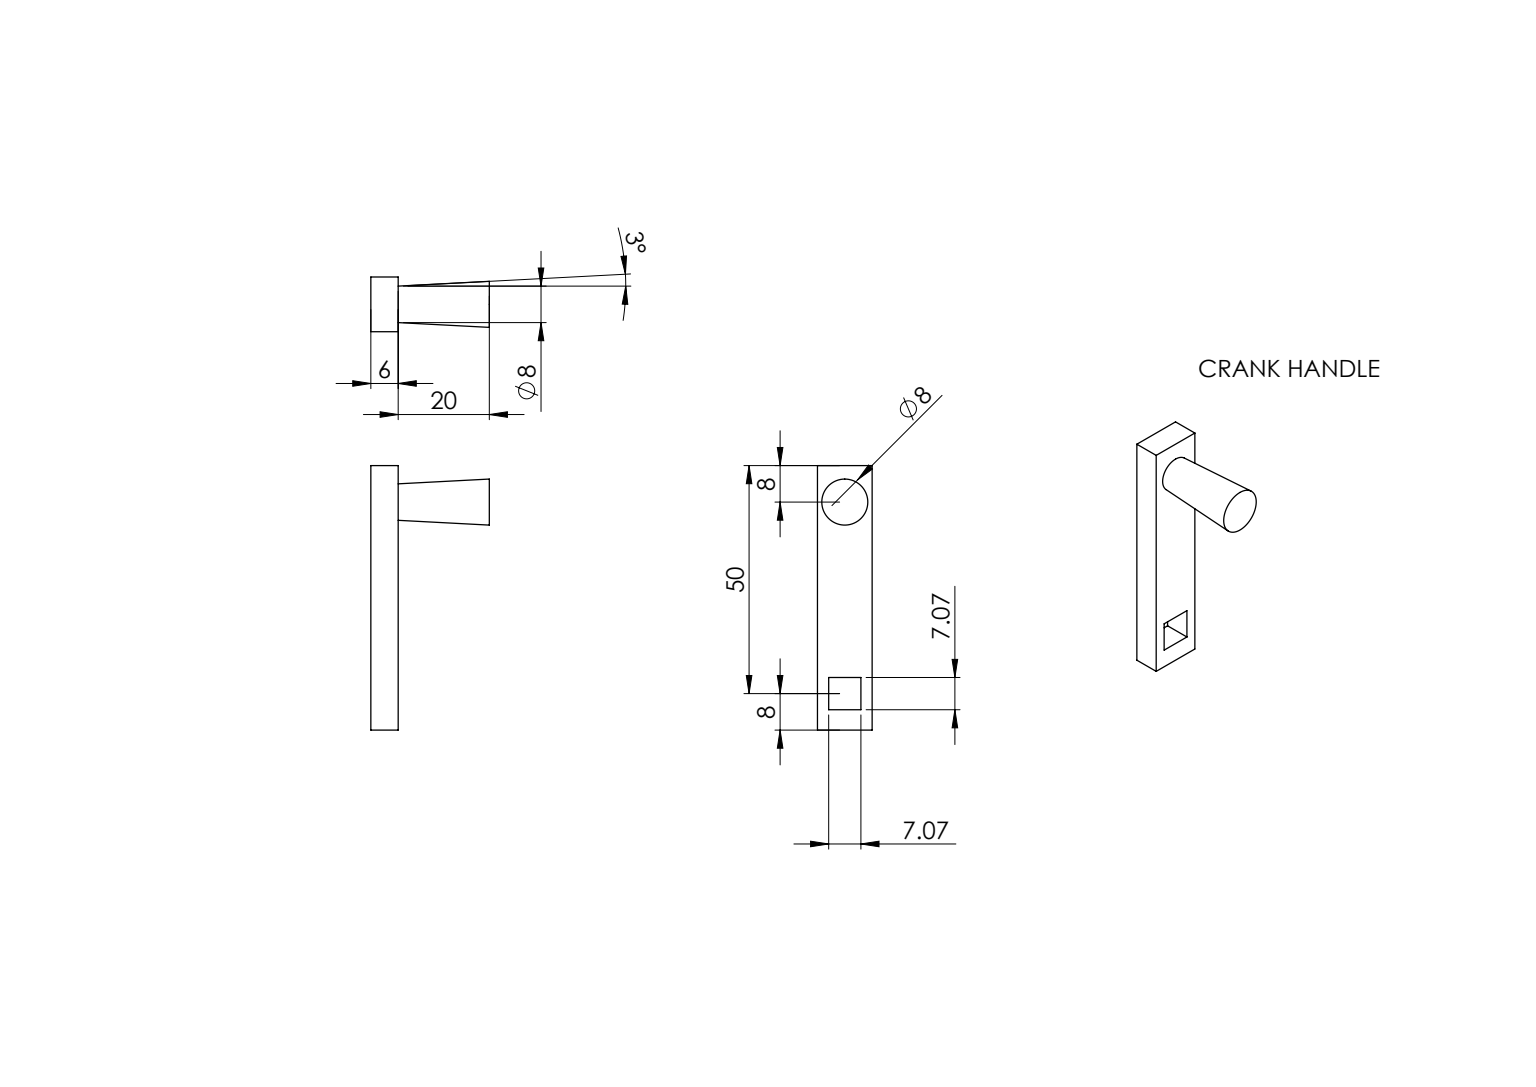
ISO-10303-21;
HEADER;
FILE_DESCRIPTION (('STEP AP214'),
    '1' );
FILE_NAME ('Crank Handle.step',
    '2026-10-22T10:02:39',
    ( '' ),
    ( '' ),
    'SwSTEP 2.0',
    'SolidWorks 2026',
    '' );
FILE_SCHEMA (( 'AUTOMOTIVE_DESIGN' ));
ENDSEC;

DATA;
#15=EDGE_LOOP ( 'NONE', ( #10379, #7375, #3120, #371 ) ) ;
#35=EDGE_CURVE ( 'NONE', #6873, #1790, #10415, .T. ) ;
#58=VECTOR ( 'NONE', #4245, 1000.000000000000000 ) ;
#60=SHAPE_DEFINITION_REPRESENTATION ( #9305, #2176 ) ;
#144=ORIENTED_EDGE ( 'NONE', *, *, #11561, .T. ) ;
#159=AXIS2_PLACEMENT_3D ( 'NONE', #745, #8186, #2789 ) ;
#163=LINE ( 'NONE', #11122, #11282 ) ;
#198=DIRECTION ( 'NONE',  ( 6.033820786006286457E-17, -1.000000000000000000, 0.000000000000000000 ) ) ;
#217=CARTESIAN_POINT ( 'NONE',  ( 47.00000000000000000, 55.00000000000000000, 6.000000000000000000 ) ) ;
#223=DIRECTION ( 'NONE',  ( -1.000000000000000000, -6.033820786006286457E-17, 0.000000000000000000 ) ) ;
#229=CARTESIAN_POINT ( 'NONE',  ( 73.00000000000000000, 91.95184441433917755, -3.614966813601447167E-16 ) ) ;
#242=DIRECTION ( 'NONE',  ( 0.000000000000000000, -0.000000000000000000, 1.000000000000000000 ) ) ;
#271=FACE_OUTER_BOUND ( 'NONE', #5676, .T. ) ;
#301=VERTEX_POINT ( 'NONE', #1190 ) ;
#315=ORIENTED_EDGE ( 'NONE', *, *, #10681, .F. ) ;
#358=ORIENTED_EDGE ( 'NONE', *, *, #7637, .F. ) ;
#371=ORIENTED_EDGE ( 'NONE', *, *, #2057, .T. ) ;
#425=ORIENTED_EDGE ( 'NONE', *, *, #6952, .F. ) ;
#440=DIRECTION ( 'NONE',  ( 0.000000000000000000, 1.000000000000000000, 0.000000000000000000 ) ) ;
#476=LINE ( 'NONE', #4199, #9328 ) ;
#477=STYLED_ITEM ( 'NONE', ( #10437 ), #9416 ) ;
#522=EDGE_CURVE ( 'NONE', #2578, #3782, #9633, .T. ) ;
#579=CARTESIAN_POINT ( 'NONE',  ( 52.99999999999999289, 58.53553390593273065, -3.535533905932738197 ) ) ;
#595=DIRECTION ( 'NONE',  ( 0.000000000000000000, 0.000000000000000000, -1.000000000000000000 ) ) ;
#645=DIRECTION ( 'NONE',  ( 0.000000000000000000, 0.000000000000000000, -1.000000000000000000 ) ) ;
#662=CARTESIAN_POINT ( 'NONE',  ( 53.00000000000000000, 47.00000000000000711, -6.000000000000000000 ) ) ;
#670=UNCERTAINTY_MEASURE_WITH_UNIT (LENGTH_MEASURE( 1.000000000000000082E-05 ), #7474, 'distance_accuracy_value', 'NONE');
#683=ORIENTED_EDGE ( 'NONE', *, *, #522, .T. ) ;
#686=CARTESIAN_POINT ( 'NONE',  ( 47.00000000000000000, 47.00000000000000711, 6.000000000000000000 ) ) ;
#697=DIRECTION ( 'NONE',  ( 0.000000000000000000, 1.000000000000000000, 0.000000000000000000 ) ) ;
#735=DIRECTION ( 'NONE',  ( -0.000000000000000000, -0.000000000000000000, 1.000000000000000000 ) ) ;
#745=CARTESIAN_POINT ( 'NONE',  ( 52.99999999999999289, 97.00000000000000000, -9.797174393178809880E-16 ) ) ;
#779=AXIS2_PLACEMENT_3D ( 'NONE', #3024, #6692, #198 ) ;
#783=( NAMED_UNIT ( * ) PLANE_ANGLE_UNIT ( ) SI_UNIT ( $, .RADIAN. ) );
#840=DIRECTION ( 'NONE',  ( -1.000000000000000000, -6.033820786006286457E-17, -0.000000000000000000 ) ) ;
#922=ORIENTED_EDGE ( 'NONE', *, *, #35, .F. ) ;
#961=VECTOR ( 'NONE', #1461, 1000.000000000000000 ) ;
#980=MANIFOLD_SOLID_BREP ( 'Cavity1', #6172 ) ;
#1018=ORIENTED_EDGE ( 'NONE', *, *, #9096, .F. ) ;
#1060=ORIENTED_EDGE ( 'NONE', *, *, #10956, .T. ) ;
#1092=EDGE_CURVE ( 'NONE', #301, #7726, #4627, .T. ) ;
#1131=ORIENTED_EDGE ( 'NONE', *, *, #4934, .T. ) ;
#1138=ORIENTED_EDGE ( 'NONE', *, *, #8425, .F. ) ;
#1145=LINE ( 'NONE', #7519, #1367 ) ;
#1176=LINE ( 'NONE', #217, #961 ) ;
#1190=CARTESIAN_POINT ( 'NONE',  ( 53.00000000000000000, 105.0000000000000142, -6.000000000000000000 ) ) ;
#1212=FACE_OUTER_BOUND ( 'NONE', #9717, .T. ) ;
#1235=( GEOMETRIC_REPRESENTATION_CONTEXT ( 3 ) GLOBAL_UNCERTAINTY_ASSIGNED_CONTEXT ( ( #3433 ) ) GLOBAL_UNIT_ASSIGNED_CONTEXT ( ( #11335, #6810, #5979 ) ) REPRESENTATION_CONTEXT ( 'NONE', 'WORKASPACE' ) );
#1280=FILL_AREA_STYLE ('',( #9367 ) ) ;
#1281=AXIS2_PLACEMENT_3D ( 'NONE', #8097, #9101, #4381 ) ;
#1335=AXIS2_PLACEMENT_3D ( 'NONE', #3104, #11347, #6769 ) ;
#1367=VECTOR ( 'NONE', #10249, 1000.000000000000000 ) ;
#1383=DIRECTION ( 'NONE',  ( 1.000000000000000000, 0.000000000000000000, 0.000000000000000000 ) ) ;
#1388=ORIENTED_EDGE ( 'NONE', *, *, #7898, .F. ) ;
#1436=DIRECTION ( 'NONE',  ( -1.000000000000000000, -6.033820786006286457E-17, -0.000000000000000000 ) ) ;
#1455=ORIENTED_EDGE ( 'NONE', *, *, #2211, .F. ) ;
#1461=DIRECTION ( 'NONE',  ( 6.033820786006286457E-17, -1.000000000000000000, 0.000000000000000000 ) ) ;
#1473=CARTESIAN_POINT ( 'NONE',  ( 53.00000000000000000, 47.00000000000000711, 0.000000000000000000 ) ) ;
#1476=ORIENTED_EDGE ( 'NONE', *, *, #6323, .T. ) ;
#1582=LINE ( 'NONE', #1637, #9387 ) ;
#1601=CARTESIAN_POINT ( 'NONE',  ( 73.00000000000000000, 97.00000000000000000, -9.797174393178809880E-16 ) ) ;
#1604=PLANE ( 'NONE',  #7645 ) ;
#1637=CARTESIAN_POINT ( 'NONE',  ( 46.99999999999999289, 58.53553390593273065, 3.535533905932731091 ) ) ;
#1734=CARTESIAN_POINT ( 'NONE',  ( 53.00000000000000000, 55.00000000000000000, -6.000000000000000000 ) ) ;
#1746=AXIS2_PLACEMENT_3D ( 'NONE', #8986, #8142, #5448 ) ;
#1756=ADVANCED_FACE ( 'NONE', ( #271 ), #4960, .T. ) ;
#1785=LINE ( 'NONE', #6246, #5721 ) ;
#1790=VERTEX_POINT ( 'NONE', #5026 ) ;
#1835=CONICAL_SURFACE ( 'NONE', #4136, 4.000000000000003553, 0.05235987755983000091 ) ;
#1840=FACE_BOUND ( 'NONE', #1900, .T. ) ;
#1843=DIRECTION ( 'NONE',  ( 6.033820786006286457E-17, -1.000000000000000000, 0.000000000000000000 ) ) ;
#1874=VERTEX_POINT ( 'NONE', #2873 ) ;
#1883=ORIENTED_EDGE ( 'NONE', *, *, #3862, .F. ) ;
#1900=EDGE_LOOP ( 'NONE', ( #3688, #6429 ) ) ;
#1905=PLANE ( 'NONE',  #9512 ) ;
#1938=VECTOR ( 'NONE', #11031, 1000.000000000000000 ) ;
#1956=DIRECTION ( 'NONE',  ( 0.000000000000000000, 1.000000000000000000, 0.000000000000000000 ) ) ;
#1967=CARTESIAN_POINT ( 'NONE',  ( 53.00000000000000000, 105.0000000000000142, 0.000000000000000000 ) ) ;
#1981=ADVANCED_FACE ( 'NONE', ( #9100 ), #7435, .T. ) ;
#2057=EDGE_CURVE ( 'NONE', #7726, #3451, #163, .T. ) ;
#2061=CARTESIAN_POINT ( 'NONE',  ( 53.00000000000000000, 105.0000000000000142, 6.000000000000000000 ) ) ;
#2146=ORIENTED_EDGE ( 'NONE', *, *, #1092, .T. ) ;
#2162=ORIENTED_EDGE ( 'NONE', *, *, #2057, .F. ) ;
#2176=SHAPE_REPRESENTATION ( 'Crank Handle', ( #4738 ), #4498 ) ;
#2211=EDGE_CURVE ( 'NONE', #3782, #1790, #1582, .T. ) ;
#2236=CARTESIAN_POINT ( 'NONE',  ( 53.00000000000000000, 55.00000000000000000, 6.000000000000000000 ) ) ;
#2267=ORIENTED_EDGE ( 'NONE', *, *, #7023, .T. ) ;
#2276=EDGE_CURVE ( 'NONE', #2578, #6873, #3915, .T. ) ;
#2281=MECHANICAL_DESIGN_GEOMETRIC_PRESENTATION_REPRESENTATION('',(#8140),#6886);
#2432=VECTOR ( 'NONE', #8895, 1000.000000000000000 ) ;
#2529=DIRECTION ( 'NONE',  ( -1.000000000000000000, -6.033820786006286457E-17, -0.000000000000000000 ) ) ;
#2576=CARTESIAN_POINT ( 'NONE',  ( 53.00000000000000000, 51.46446609406726935, -3.535533905932738197 ) ) ;
#2578=VERTEX_POINT ( 'NONE', #6201 ) ;
#2622=VECTOR ( 'NONE', #2700, 1000.000000000000114 ) ;
#2666=ORIENTED_EDGE ( 'NONE', *, *, #10956, .F. ) ;
#2680=ORIENTED_EDGE ( 'NONE', *, *, #10681, .T. ) ;
#2697=CARTESIAN_POINT ( 'NONE',  ( 47.00000000000000000, 105.0000000000000142, 0.000000000000000000 ) ) ;
#2700=DIRECTION ( 'NONE',  ( 0.9986295347545739443, 0.05233595624294401505, 0.000000000000000000 ) ) ;
#2748=DIRECTION ( 'NONE',  ( 1.000000000000000000, 6.033820786006286457E-17, 0.000000000000000000 ) ) ;
#2774=EDGE_CURVE ( 'NONE', #9261, #3782, #8383, .T. ) ;
#2789=DIRECTION ( 'NONE',  ( 0.000000000000000000, 1.000000000000000000, 0.000000000000000000 ) ) ;
#2864=AXIS2_PLACEMENT_3D ( 'NONE', #1601, #5268, #697 ) ;
#2870=UNCERTAINTY_MEASURE_WITH_UNIT (LENGTH_MEASURE( 1.000000000000000082E-05 ), #9951, 'distance_accuracy_value', 'NONE');
#2873=CARTESIAN_POINT ( 'NONE',  ( 53.00000000000000000, 51.46446609406726935, 3.535533905932731091 ) ) ;
#2938=ORIENTED_EDGE ( 'NONE', *, *, #6952, .T. ) ;
#3024=CARTESIAN_POINT ( 'NONE',  ( 47.00000000000000000, 2.835895769422954721E-15, 0.000000000000000000 ) ) ;
#3026=SHAPE_REPRESENTATION_RELATIONSHIP ( 'NONE' , 'NONE' ,  #2176, #9416 ) ;
#3080=EDGE_LOOP ( 'NONE', ( #5000, #1476 ) ) ;
#3087=VECTOR ( 'NONE', #2529, 1000.000000000000000 ) ;
#3104=CARTESIAN_POINT ( 'NONE',  ( 53.00000000000000000, 51.46446609406726935, -3.535533905932738197 ) ) ;
#3120=ORIENTED_EDGE ( 'NONE', *, *, #5936, .F. ) ;
#3146=FACE_OUTER_BOUND ( 'NONE', #15, .T. ) ;
#3211=FACE_OUTER_BOUND ( 'NONE', #5333, .T. ) ;
#3280=VERTEX_POINT ( 'NONE', #686 ) ;
#3289=EDGE_LOOP ( 'NONE', ( #1388, #922, #144, #8606 ) ) ;
#3293=VERTEX_POINT ( 'NONE', #8010 ) ;
#3296=CARTESIAN_POINT ( 'NONE',  ( 47.00000000000000000, 51.46446609406726935, -3.535533905932738197 ) ) ;
#3313=CARTESIAN_POINT ( 'NONE',  ( 52.99999999999999289, 93.00000000000000000, -4.256777005095426300E-16 ) ) ;
#3334=CARTESIAN_POINT ( 'NONE',  ( 53.00000000000000000, 47.00000000000000711, 6.000000000000000000 ) ) ;
#3433=UNCERTAINTY_MEASURE_WITH_UNIT (LENGTH_MEASURE( 1.000000000000000082E-05 ), #11335, 'distance_accuracy_value', 'NONE');
#3451=VERTEX_POINT ( 'NONE', #7408 ) ;
#3536=ORIENTED_EDGE ( 'NONE', *, *, #9673, .F. ) ;
#3553=CARTESIAN_POINT ( 'NONE',  ( 53.00000000000000000, 105.0000000000000142, 0.000000000000000000 ) ) ;
#3576=VECTOR ( 'NONE', #10475, 1000.000000000000000 ) ;
#3581=ADVANCED_FACE ( 'NONE', ( #4830 ), #1835, .T. ) ;
#3611=CARTESIAN_POINT ( 'NONE',  ( 53.00000000000000000, 51.46446609406726935, -3.535533905932738197 ) ) ;
#3654=DIRECTION ( 'NONE',  ( 0.000000000000000000, 0.000000000000000000, -1.000000000000000000 ) ) ;
#3688=ORIENTED_EDGE ( 'NONE', *, *, #4934, .F. ) ;
#3759=CARTESIAN_POINT ( 'NONE',  ( 53.00000000000000000, 47.00000000000000711, 0.000000000000000000 ) ) ;
#3762=FACE_OUTER_BOUND ( 'NONE', #7978, .T. ) ;
#3782=VERTEX_POINT ( 'NONE', #7109 ) ;
#3862=EDGE_CURVE ( 'NONE', #3293, #9431, #1145, .T. ) ;
#3915=LINE ( 'NONE', #7523, #8630 ) ;
#3922=DIRECTION ( 'NONE',  ( 1.000000000000000000, 6.033820786006286457E-17, 0.000000000000000000 ) ) ;
#3985=( NAMED_UNIT ( * ) SI_UNIT ( $, .STERADIAN. ) SOLID_ANGLE_UNIT ( ) );
#4004=CARTESIAN_POINT ( 'NONE',  ( 53.00000000000000000, 55.00000000000000000, -6.000000000000000000 ) ) ;
#4032=PRODUCT_DEFINITION ( 'UNKNOWN', '', #9471, #10598 ) ;
#4045=FACE_OUTER_BOUND ( 'NONE', #6490, .T. ) ;
#4080=CARTESIAN_POINT ( 'NONE',  ( 53.00000000000000000, 51.46446609406726935, 3.535533905932731091 ) ) ;
#4136=AXIS2_PLACEMENT_3D ( 'NONE', #8661, #3922, #9490 ) ;
#4199=CARTESIAN_POINT ( 'NONE',  ( 47.00000000000000000, 47.00000000000000711, 0.000000000000000000 ) ) ;
#4239=LINE ( 'NONE', #3334, #5310 ) ;
#4245=DIRECTION ( 'NONE',  ( -1.000000000000000000, -6.033820786006286457E-17, -0.000000000000000000 ) ) ;
#4257=LINE ( 'NONE', #4080, #3576 ) ;
#4297=ORIENTED_EDGE ( 'NONE', *, *, #6682, .F. ) ;
#4306=DIRECTION ( 'NONE',  ( -1.000000000000000000, 0.000000000000000000, -0.000000000000000000 ) ) ;
#4315=DIRECTION ( 'NONE',  ( 0.000000000000000000, -0.000000000000000000, 1.000000000000000000 ) ) ;
#4321=ORIENTED_EDGE ( 'NONE', *, *, #2774, .T. ) ;
#4351=ORIENTED_EDGE ( 'NONE', *, *, #6323, .F. ) ;
#4356=CIRCLE ( 'NONE', #1281, 4.000000000000003553 ) ;
#4381=DIRECTION ( 'NONE',  ( 0.000000000000000000, 1.000000000000000000, 0.000000000000000000 ) ) ;
#4445=CONICAL_SURFACE ( 'NONE', #9212, 4.000000000000003553, 0.05235987755983000091 ) ;
#4448=LINE ( 'NONE', #9765, #3087 ) ;
#4464=ORIENTED_EDGE ( 'NONE', *, *, #3862, .T. ) ;
#4466=ADVANCED_FACE ( 'NONE', ( #9871 ), #6242, .T. ) ;
#4495=PLANE ( 'NONE',  #10458 ) ;
#4498=( GEOMETRIC_REPRESENTATION_CONTEXT ( 3 ) GLOBAL_UNCERTAINTY_ASSIGNED_CONTEXT ( ( #670 ) ) GLOBAL_UNIT_ASSIGNED_CONTEXT ( ( #7474, #6756, #3985 ) ) REPRESENTATION_CONTEXT ( 'NONE', 'WORKASPACE' ) );
#4554=CARTESIAN_POINT ( 'NONE',  ( 52.99999999999999289, 58.53553390593273065, 3.535533905932731091 ) ) ;
#4556=LINE ( 'NONE', #9159, #2622 ) ;
#4574=PRODUCT_CONTEXT ( 'NONE', #10659, 'mechanical' ) ;
#4604=VECTOR ( 'NONE', #11137, 1000.000000000000000 ) ;
#4627=LINE ( 'NONE', #3553, #7837 ) ;
#4655=VERTEX_POINT ( 'NONE', #2576 ) ;
#4702=EDGE_CURVE ( 'NONE', #10425, #9224, #9449, .T. ) ;
#4738=AXIS2_PLACEMENT_3D ( 'NONE', #6164, #8011, #1383 ) ;
#4756=PLANE ( 'NONE',  #7042 ) ;
#4830=FACE_OUTER_BOUND ( 'NONE', #6926, .T. ) ;
#4852=EDGE_LOOP ( 'NONE', ( #1455, #9924, #5836, #11754 ) ) ;
#4933=EDGE_LOOP ( 'NONE', ( #2666, #7561, #5617, #4351 ) ) ;
#4934=EDGE_CURVE ( 'NONE', #9462, #10179, #10101, .T. ) ;
#4960=PLANE ( 'NONE',  #1335 ) ;
#5000=ORIENTED_EDGE ( 'NONE', *, *, #7637, .T. ) ;
#5026=CARTESIAN_POINT ( 'NONE',  ( 46.99999999999999289, 58.53553390593273065, 3.535533905932731091 ) ) ;
#5076=ORIENTED_EDGE ( 'NONE', *, *, #10514, .F. ) ;
#5082=ORIENTED_EDGE ( 'NONE', *, *, #9241, .T. ) ;
#5161=LINE ( 'NONE', #10593, #7883 ) ;
#5232=ORIENTED_EDGE ( 'NONE', *, *, #2211, .T. ) ;
#5268=DIRECTION ( 'NONE',  ( 1.000000000000000000, 6.033820786006286457E-17, 0.000000000000000000 ) ) ;
#5310=VECTOR ( 'NONE', #11588, 1000.000000000000000 ) ;
#5331=VECTOR ( 'NONE', #9283, 1000.000000000000000 ) ;
#5333=EDGE_LOOP ( 'NONE', ( #2680, #1018, #8123, #6213 ) ) ;
#5338=DIRECTION ( 'NONE',  ( 0.9986295347545739443, -0.05233595624294389015, 6.409306129323724811E-18 ) ) ;
#5448=DIRECTION ( 'NONE',  ( -6.033820786006286457E-17, 1.000000000000000000, 0.000000000000000000 ) ) ;
#5457=ORIENTED_EDGE ( 'NONE', *, *, #7340, .F. ) ;
#5486=AXIS2_PLACEMENT_3D ( 'NONE', #10165, #223, #6595 ) ;
#5586=ADVANCED_FACE ( 'NONE', ( #8808 ), #1604, .T. ) ;
#5617=ORIENTED_EDGE ( 'NONE', *, *, #11056, .T. ) ;
#5637=DIRECTION ( 'NONE',  ( 0.000000000000000000, -1.000000000000000000, 0.000000000000000000 ) ) ;
#5676=EDGE_LOOP ( 'NONE', ( #5932, #425, #6634, #683 ) ) ;
#5721=VECTOR ( 'NONE', #5338, 1000.000000000000114 ) ;
#5726=ADVANCED_FACE ( 'NONE', ( #3211 ), #9563, .F. ) ;
#5772=CARTESIAN_POINT ( 'NONE',  ( 53.00000000000000000, 47.00000000000000711, 6.000000000000000000 ) ) ;
#5793=APPLICATION_CONTEXT ( 'automotive_design' ) ;
#5836=ORIENTED_EDGE ( 'NONE', *, *, #2276, .T. ) ;
#5905=DIRECTION ( 'NONE',  ( 6.033820786006286457E-17, -1.000000000000000000, 0.000000000000000000 ) ) ;
#5912=CARTESIAN_POINT ( 'NONE',  ( 53.00000000000000000, 55.00000000000000000, 6.000000000000000000 ) ) ;
#5924=ORIENTED_EDGE ( 'NONE', *, *, #1092, .F. ) ;
#5932=ORIENTED_EDGE ( 'NONE', *, *, #2774, .F. ) ;
#5936=EDGE_CURVE ( 'NONE', #7726, #10425, #11332, .T. ) ;
#5963=AXIS2_PLACEMENT_3D ( 'NONE', #4554, #1843, #10104 ) ;
#5979=( NAMED_UNIT ( * ) SI_UNIT ( $, .STERADIAN. ) SOLID_ANGLE_UNIT ( ) );
#5988=DIRECTION ( 'NONE',  ( -0.000000000000000000, 1.000000000000000000, 0.000000000000000000 ) ) ;
#6018=ORIENTED_EDGE ( 'NONE', *, *, #9096, .T. ) ;
#6083=AXIS2_PLACEMENT_3D ( 'NONE', #5912, #9616, #11391 ) ;
#6093=PLANE ( 'NONE',  #6083 ) ;
#6164=CARTESIAN_POINT ( 'NONE',  ( 0.000000000000000000, 0.000000000000000000, 0.000000000000000000 ) ) ;
#6172=CLOSED_SHELL ( 'NONE', ( #3581, #9537, #7863, #5726, #11146, #11392, #11532, #7975, #4466, #1756, #1981, #5586, #10100 ) ) ;
#6189=LINE ( 'NONE', #2697, #7815 ) ;
#6201=CARTESIAN_POINT ( 'NONE',  ( 52.99999999999999289, 58.53553390593273065, -3.535533905932738197 ) ) ;
#6213=ORIENTED_EDGE ( 'NONE', *, *, #9946, .T. ) ;
#6242=PLANE ( 'NONE',  #1746 ) ;
#6246=CARTESIAN_POINT ( 'NONE',  ( 52.99999999999999289, 93.00000000000000000, -4.898587196589397051E-16 ) ) ;
#6279=ORIENTED_EDGE ( 'NONE', *, *, #9241, .F. ) ;
#6323=EDGE_CURVE ( 'NONE', #11278, #6597, #8037, .T. ) ;
#6396=ORIENTED_EDGE ( 'NONE', *, *, #2276, .F. ) ;
#6429=ORIENTED_EDGE ( 'NONE', *, *, #11121, .F. ) ;
#6474=FACE_BOUND ( 'NONE', #8910, .T. ) ;
#6490=EDGE_LOOP ( 'NONE', ( #315, #4297, #11515, #4464 ) ) ;
#6531=DIRECTION ( 'NONE',  ( 0.000000000000000000, 0.000000000000000000, -1.000000000000000000 ) ) ;
#6595=DIRECTION ( 'NONE',  ( 6.033820786006286457E-17, -1.000000000000000000, 0.000000000000000000 ) ) ;
#6597=VERTEX_POINT ( 'NONE', #7541 ) ;
#6634=ORIENTED_EDGE ( 'NONE', *, *, #10514, .T. ) ;
#6682=EDGE_CURVE ( 'NONE', #3451, #3280, #1176, .T. ) ;
#6692=DIRECTION ( 'NONE',  ( -1.000000000000000000, -6.033820786006286457E-17, 0.000000000000000000 ) ) ;
#6734=CARTESIAN_POINT ( 'NONE',  ( 53.00000000000000000, 51.46446609406726935, -3.535533905932738197 ) ) ;
#6754=FACE_BOUND ( 'NONE', #7352, .T. ) ;
#6756=( NAMED_UNIT ( * ) PLANE_ANGLE_UNIT ( ) SI_UNIT ( $, .RADIAN. ) );
#6769=DIRECTION ( 'NONE',  ( 1.000000000000000000, 0.000000000000000000, -0.000000000000000000 ) ) ;
#6774=DIRECTION ( 'NONE',  ( 6.033820786006286457E-17, -1.000000000000000000, 0.000000000000000000 ) ) ;
#6810=( NAMED_UNIT ( * ) PLANE_ANGLE_UNIT ( ) SI_UNIT ( $, .RADIAN. ) );
#6824=ORIENTED_EDGE ( 'NONE', *, *, #5936, .T. ) ;
#6873=VERTEX_POINT ( 'NONE', #8113 ) ;
#6886=( GEOMETRIC_REPRESENTATION_CONTEXT ( 3 ) GLOBAL_UNCERTAINTY_ASSIGNED_CONTEXT ( ( #2870 ) ) GLOBAL_UNIT_ASSIGNED_CONTEXT ( ( #9951, #783, #10848 ) ) REPRESENTATION_CONTEXT ( 'NONE', 'WORKASPACE' ) );
#6926=EDGE_LOOP ( 'NONE', ( #1131, #1060, #358, #11714 ) ) ;
#6941=DIRECTION ( 'NONE',  ( 0.000000000000000000, -0.000000000000000000, 1.000000000000000000 ) ) ;
#6952=EDGE_CURVE ( 'NONE', #4655, #9261, #8226, .T. ) ;
#7023=EDGE_CURVE ( 'NONE', #8687, #9261, #7335, .T. ) ;
#7042=AXIS2_PLACEMENT_3D ( 'NONE', #9422, #9482, #10197 ) ;
#7045=ORIENTED_EDGE ( 'NONE', *, *, #10885, .T. ) ;
#7092=VECTOR ( 'NONE', #5905, 1000.000000000000000 ) ;
#7109=CARTESIAN_POINT ( 'NONE',  ( 47.00000000000000000, 58.53553390593273065, -3.535533905932743526 ) ) ;
#7297=VECTOR ( 'NONE', #10351, 1000.000000000000000 ) ;
#7335=LINE ( 'NONE', #10008, #4604 ) ;
#7340=EDGE_CURVE ( 'NONE', #1874, #8687, #4448, .T. ) ;
#7352=EDGE_LOOP ( 'NONE', ( #2267, #4321, #5232, #10966 ) ) ;
#7375=ORIENTED_EDGE ( 'NONE', *, *, #9946, .F. ) ;
#7403=PRODUCT ( 'Crank Handle', 'Crank Handle', '', ( #4574 ) ) ;
#7408=CARTESIAN_POINT ( 'NONE',  ( 47.00000000000000000, 105.0000000000000142, 6.000000000000000000 ) ) ;
#7435=PLANE ( 'NONE',  #5963 ) ;
#7474=( LENGTH_UNIT ( ) NAMED_UNIT ( * ) SI_UNIT ( .MILLI., .METRE. ) );
#7499=DIRECTION ( 'NONE',  ( 0.000000000000000000, 0.000000000000000000, -1.000000000000000000 ) ) ;
#7511=LINE ( 'NONE', #6734, #5331 ) ;
#7519=CARTESIAN_POINT ( 'NONE',  ( 47.00000000000000000, 55.00000000000000000, -6.000000000000000000 ) ) ;
#7523=CARTESIAN_POINT ( 'NONE',  ( 52.99999999999999289, 58.53553390593273065, 3.535533905932731091 ) ) ;
#7541=CARTESIAN_POINT ( 'NONE',  ( 73.00000000000000000, 102.0481555856608225, -9.797174393178809880E-16 ) ) ;
#7561=ORIENTED_EDGE ( 'NONE', *, *, #11121, .T. ) ;
#7585=PLANE ( 'NONE',  #779 ) ;
#7633=CARTESIAN_POINT ( 'NONE',  ( 47.00000000000000711, 51.46446609406725514, 3.535533905932731091 ) ) ;
#7637=EDGE_CURVE ( 'NONE', #6597, #11278, #10149, .T. ) ;
#7645=AXIS2_PLACEMENT_3D ( 'NONE', #10703, #645, #4306 ) ;
#7726=VERTEX_POINT ( 'NONE', #2061 ) ;
#7815=VECTOR ( 'NONE', #4315, 1000.000000000000000 ) ;
#7821=ORIENTED_EDGE ( 'NONE', *, *, #4702, .T. ) ;
#7824=EDGE_LOOP ( 'NONE', ( #1883, #1138, #9985, #6018 ) ) ;
#7837=VECTOR ( 'NONE', #242, 1000.000000000000000 ) ;
#7860=DIRECTION ( 'NONE',  ( -1.000000000000000000, -0.000000000000000000, -0.000000000000000000 ) ) ;
#7863=ADVANCED_FACE ( 'NONE', ( #6754, #4045 ), #7585, .T. ) ;
#7883=VECTOR ( 'NONE', #7860, 1000.000000000000000 ) ;
#7898=EDGE_CURVE ( 'NONE', #1790, #8687, #11149, .T. ) ;
#7975=ADVANCED_FACE ( 'NONE', ( #10494 ), #4445, .T. ) ;
#7978=EDGE_LOOP ( 'NONE', ( #7821, #3536, #2146, #6824 ) ) ;
#8010=CARTESIAN_POINT ( 'NONE',  ( 47.00000000000000000, 105.0000000000000142, -6.000000000000000000 ) ) ;
#8011=DIRECTION ( 'NONE',  ( 0.000000000000000000, 0.000000000000000000, 1.000000000000000000 ) ) ;
#8037=CIRCLE ( 'NONE', #2864, 5.048155585660824229 ) ;
#8097=CARTESIAN_POINT ( 'NONE',  ( 52.99999999999999289, 97.00000000000000000, -9.797174393178809880E-16 ) ) ;
#8113=CARTESIAN_POINT ( 'NONE',  ( 52.99999999999999289, 58.53553390593273065, 3.535533905932731091 ) ) ;
#8123=ORIENTED_EDGE ( 'NONE', *, *, #4702, .F. ) ;
#8140=STYLED_ITEM('',(#11874),#980);
#8142=DIRECTION ( 'NONE',  ( 1.000000000000000000, 6.033820786006286457E-17, 0.000000000000000000 ) ) ;
#8186=DIRECTION ( 'NONE',  ( 1.000000000000000000, 6.033820786006286457E-17, 0.000000000000000000 ) ) ;
#8226=LINE ( 'NONE', #3611, #10928 ) ;
#8383=LINE ( 'NONE', #8624, #7297 ) ;
#8397=ORIENTED_EDGE ( 'NONE', *, *, #11561, .F. ) ;
#8420=EDGE_LOOP ( 'NONE', ( #7045, #2162, #5924, #9018 ) ) ;
#8425=EDGE_CURVE ( 'NONE', #301, #3293, #5161, .T. ) ;
#8459=VECTOR ( 'NONE', #1436, 1000.000000000000000 ) ;
#8501=ORIENTED_EDGE ( 'NONE', *, *, #7023, .F. ) ;
#8518=COLOUR_RGB ( '',0.8941176470588234615, 0.8941176470588234615, 0.8941176470588234615 ) ;
#8606=ORIENTED_EDGE ( 'NONE', *, *, #7340, .T. ) ;
#8624=CARTESIAN_POINT ( 'NONE',  ( 47.00000000000000000, 51.46446609406726935, -3.535533905932738197 ) ) ;
#8630=VECTOR ( 'NONE', #11144, 1000.000000000000000 ) ;
#8661=CARTESIAN_POINT ( 'NONE',  ( 52.99999999999999289, 97.00000000000000000, -9.797174393178809880E-16 ) ) ;
#8687=VERTEX_POINT ( 'NONE', #7633 ) ;
#8717=LINE ( 'NONE', #9670, #2432 ) ;
#8748=VECTOR ( 'NONE', #11622, 1000.000000000000000 ) ;
#8808=FACE_OUTER_BOUND ( 'NONE', #3289, .T. ) ;
#8883=LINE ( 'NONE', #662, #8748 ) ;
#8895=DIRECTION ( 'NONE',  ( 9.813077866773612233E-16, -1.000000000000000000, -0.000000000000000000 ) ) ;
#8910=EDGE_LOOP ( 'NONE', ( #5076, #6279, #8397, #6396 ) ) ;
#8986=CARTESIAN_POINT ( 'NONE',  ( 73.00000000000000000, 97.00000000000000000, -9.797174393178809880E-16 ) ) ;
#9018=ORIENTED_EDGE ( 'NONE', *, *, #8425, .T. ) ;
#9096=EDGE_CURVE ( 'NONE', #9224, #9431, #8883, .T. ) ;
#9100=FACE_OUTER_BOUND ( 'NONE', #4852, .T. ) ;
#9101=DIRECTION ( 'NONE',  ( 1.000000000000000000, 6.033820786006286457E-17, 0.000000000000000000 ) ) ;
#9130=VECTOR ( 'NONE', #6774, 1000.000000000000000 ) ;
#9159=CARTESIAN_POINT ( 'NONE',  ( 52.99999999999999289, 101.0000000000000000, -9.797174393178809880E-16 ) ) ;
#9212=AXIS2_PLACEMENT_3D ( 'NONE', #11511, #10670, #440 ) ;
#9224=VERTEX_POINT ( 'NONE', #11074 ) ;
#9241=EDGE_CURVE ( 'NONE', #1874, #4655, #4257, .T. ) ;
#9261=VERTEX_POINT ( 'NONE', #3296 ) ;
#9283=DIRECTION ( 'NONE',  ( -9.813077866773612233E-16, 1.000000000000000000, 0.000000000000000000 ) ) ;
#9305=PRODUCT_DEFINITION_SHAPE ( 'NONE', 'NONE',  #4032 ) ;
#9328=VECTOR ( 'NONE', #595, 1000.000000000000000 ) ;
#9367=FILL_AREA_STYLE_COLOUR ( '', #8518 ) ;
#9387=VECTOR ( 'NONE', #735, 1000.000000000000000 ) ;
#9389=AXIS2_PLACEMENT_3D ( 'NONE', #11051, #2748, #1956 ) ;
#9416=ADVANCED_BREP_SHAPE_REPRESENTATION ( '', ( #980, #4738 ), #4498 ) ;
#9422=CARTESIAN_POINT ( 'NONE',  ( 53.00000000000000000, 51.46446609406726935, 3.535533905932731091 ) ) ;
#9429=SURFACE_STYLE_FILL_AREA ( #1280 ) ;
#9431=VERTEX_POINT ( 'NONE', #11486 ) ;
#9449=LINE ( 'NONE', #3759, #10921 ) ;
#9462=VERTEX_POINT ( 'NONE', #10645 ) ;
#9471=PRODUCT_DEFINITION_FORMATION_WITH_SPECIFIED_SOURCE ( 'ANY', '', #7403, .NOT_KNOWN. ) ;
#9482=DIRECTION ( 'NONE',  ( -6.033820786006286457E-17, 1.000000000000000000, 0.000000000000000000 ) ) ;
#9488=CARTESIAN_POINT ( 'NONE',  ( 47.00000000000000000, 51.46446609406726935, 3.535533905932731091 ) ) ;
#9490=DIRECTION ( 'NONE',  ( 0.000000000000000000, 1.000000000000000000, 0.000000000000000000 ) ) ;
#9512=AXIS2_PLACEMENT_3D ( 'NONE', #1967, #5637, #7499 ) ;
#9537=ADVANCED_FACE ( 'NONE', ( #3762, #1840, #6474 ), #10286, .F. ) ;
#9553=AXIS2_PLACEMENT_3D ( 'NONE', #1473, #5988, #6941 ) ;
#9563=PLANE ( 'NONE',  #9553 ) ;
#9616=DIRECTION ( 'NONE',  ( 0.000000000000000000, 0.000000000000000000, -1.000000000000000000 ) ) ;
#9633=LINE ( 'NONE', #579, #58 ) ;
#9670=CARTESIAN_POINT ( 'NONE',  ( 53.00000000000000000, 51.46446609406726935, 3.535533905932731091 ) ) ;
#9673=EDGE_CURVE ( 'NONE', #301, #9224, #10942, .T. ) ;
#9717=EDGE_LOOP ( 'NONE', ( #8501, #5457, #5082, #2938 ) ) ;
#9765=CARTESIAN_POINT ( 'NONE',  ( 53.00000000000000000, 51.46446609406726935, 3.535533905932731091 ) ) ;
#9849=MECHANICAL_DESIGN_GEOMETRIC_PRESENTATION_REPRESENTATION('',(#477),#1235);
#9871=FACE_OUTER_BOUND ( 'NONE', #3080, .T. ) ;
#9924=ORIENTED_EDGE ( 'NONE', *, *, #522, .F. ) ;
#9946=EDGE_CURVE ( 'NONE', #10425, #3280, #4239, .T. ) ;
#9951=( LENGTH_UNIT ( ) NAMED_UNIT ( * ) SI_UNIT ( .MILLI., .METRE. ) );
#9985=ORIENTED_EDGE ( 'NONE', *, *, #9673, .T. ) ;
#10008=CARTESIAN_POINT ( 'NONE',  ( 47.00000000000000000, 51.46446609406726935, 3.535533905932731091 ) ) ;
#10100=ADVANCED_FACE ( 'NONE', ( #1212 ), #4756, .T. ) ;
#10101=CIRCLE ( 'NONE', #159, 4.000000000000003553 ) ;
#10104=DIRECTION ( 'NONE',  ( 1.000000000000000000, 6.033820786006286457E-17, 0.000000000000000000 ) ) ;
#10105=FACE_OUTER_BOUND ( 'NONE', #8420, .T. ) ;
#10149=CIRCLE ( 'NONE', #9389, 5.048155585660824229 ) ;
#10165=CARTESIAN_POINT ( 'NONE',  ( 53.00000000000000000, 2.835895769422954721E-15, 0.000000000000000000 ) ) ;
#10179=VERTEX_POINT ( 'NONE', #3313 ) ;
#10197=DIRECTION ( 'NONE',  ( -1.000000000000000000, -6.033820786006286457E-17, 0.000000000000000000 ) ) ;
#10249=DIRECTION ( 'NONE',  ( 6.033820786006286457E-17, -1.000000000000000000, 0.000000000000000000 ) ) ;
#10263=SURFACE_STYLE_USAGE ( .BOTH. , #10326 ) ;
#10286=PLANE ( 'NONE',  #5486 ) ;
#10326=SURFACE_SIDE_STYLE ('',( #9429 ) ) ;
#10351=DIRECTION ( 'NONE',  ( -9.813077866773612233E-16, 1.000000000000000000, 0.000000000000000000 ) ) ;
#10379=ORIENTED_EDGE ( 'NONE', *, *, #6682, .T. ) ;
#10415=LINE ( 'NONE', #11423, #8459 ) ;
#10425=VERTEX_POINT ( 'NONE', #5772 ) ;
#10437=PRESENTATION_STYLE_ASSIGNMENT (( #10263 ) ) ;
#10458=AXIS2_PLACEMENT_3D ( 'NONE', #1734, #3654, #11788 ) ;
#10475=DIRECTION ( 'NONE',  ( 0.000000000000000000, 0.000000000000000000, -1.000000000000000000 ) ) ;
#10494=FACE_OUTER_BOUND ( 'NONE', #4933, .T. ) ;
#10514=EDGE_CURVE ( 'NONE', #4655, #2578, #7511, .T. ) ;
#10593=CARTESIAN_POINT ( 'NONE',  ( 53.00000000000000000, 105.0000000000000142, -6.000000000000000000 ) ) ;
#10598=PRODUCT_DEFINITION_CONTEXT ( 'detailed design', #5793, 'design' ) ;
#10645=CARTESIAN_POINT ( 'NONE',  ( 52.99999999999999289, 101.0000000000000000, -9.797174393178809880E-16 ) ) ;
#10659=APPLICATION_CONTEXT ( 'automotive_design' ) ;
#10670=DIRECTION ( 'NONE',  ( 1.000000000000000000, 6.033820786006286457E-17, 0.000000000000000000 ) ) ;
#10681=EDGE_CURVE ( 'NONE', #3280, #9431, #476, .T. ) ;
#10703=CARTESIAN_POINT ( 'NONE',  ( 53.00000000000000000, 51.46446609406726935, 3.535533905932731091 ) ) ;
#10848=( NAMED_UNIT ( * ) SI_UNIT ( $, .STERADIAN. ) SOLID_ANGLE_UNIT ( ) );
#10885=EDGE_CURVE ( 'NONE', #3293, #3451, #6189, .T. ) ;
#10890=FACE_OUTER_BOUND ( 'NONE', #7824, .T. ) ;
#10921=VECTOR ( 'NONE', #6531, 1000.000000000000000 ) ;
#10928=VECTOR ( 'NONE', #840, 1000.000000000000000 ) ;
#10942=LINE ( 'NONE', #4004, #9130 ) ;
#10956=EDGE_CURVE ( 'NONE', #10179, #11278, #1785, .T. ) ;
#10966=ORIENTED_EDGE ( 'NONE', *, *, #7898, .T. ) ;
#11031=DIRECTION ( 'NONE',  ( 9.813077866773612233E-16, -1.000000000000000000, -0.000000000000000000 ) ) ;
#11051=CARTESIAN_POINT ( 'NONE',  ( 73.00000000000000000, 97.00000000000000000, -9.797174393178809880E-16 ) ) ;
#11056=EDGE_CURVE ( 'NONE', #9462, #6597, #4556, .T. ) ;
#11074=CARTESIAN_POINT ( 'NONE',  ( 53.00000000000000000, 47.00000000000000711, -6.000000000000000000 ) ) ;
#11121=EDGE_CURVE ( 'NONE', #10179, #9462, #4356, .T. ) ;
#11122=CARTESIAN_POINT ( 'NONE',  ( 53.00000000000000000, 105.0000000000000142, 6.000000000000000000 ) ) ;
#11137=DIRECTION ( 'NONE',  ( 0.000000000000000000, 0.000000000000000000, -1.000000000000000000 ) ) ;
#11144=DIRECTION ( 'NONE',  ( -0.000000000000000000, -0.000000000000000000, 1.000000000000000000 ) ) ;
#11146=ADVANCED_FACE ( 'NONE', ( #10890 ), #4495, .T. ) ;
#11149=LINE ( 'NONE', #9488, #1938 ) ;
#11278=VERTEX_POINT ( 'NONE', #229 ) ;
#11282=VECTOR ( 'NONE', #11312, 1000.000000000000000 ) ;
#11312=DIRECTION ( 'NONE',  ( -1.000000000000000000, -0.000000000000000000, -0.000000000000000000 ) ) ;
#11332=LINE ( 'NONE', #2236, #7092 ) ;
#11335=( LENGTH_UNIT ( ) NAMED_UNIT ( * ) SI_UNIT ( .MILLI., .METRE. ) );
#11347=DIRECTION ( 'NONE',  ( 0.000000000000000000, -0.000000000000000000, 1.000000000000000000 ) ) ;
#11391=DIRECTION ( 'NONE',  ( -1.000000000000000000, 0.000000000000000000, -0.000000000000000000 ) ) ;
#11392=ADVANCED_FACE ( 'NONE', ( #10105 ), #1905, .F. ) ;
#11423=CARTESIAN_POINT ( 'NONE',  ( 52.99999999999999289, 58.53553390593273065, 3.535533905932731091 ) ) ;
#11486=CARTESIAN_POINT ( 'NONE',  ( 47.00000000000000000, 47.00000000000000711, -6.000000000000000000 ) ) ;
#11511=CARTESIAN_POINT ( 'NONE',  ( 52.99999999999999289, 97.00000000000000000, -9.797174393178809880E-16 ) ) ;
#11515=ORIENTED_EDGE ( 'NONE', *, *, #10885, .F. ) ;
#11532=ADVANCED_FACE ( 'NONE', ( #3146 ), #6093, .F. ) ;
#11561=EDGE_CURVE ( 'NONE', #6873, #1874, #8717, .T. ) ;
#11588=DIRECTION ( 'NONE',  ( -1.000000000000000000, -0.000000000000000000, -0.000000000000000000 ) ) ;
#11622=DIRECTION ( 'NONE',  ( -1.000000000000000000, -0.000000000000000000, -0.000000000000000000 ) ) ;
#11714=ORIENTED_EDGE ( 'NONE', *, *, #11056, .F. ) ;
#11754=ORIENTED_EDGE ( 'NONE', *, *, #35, .T. ) ;
#11788=DIRECTION ( 'NONE',  ( -1.000000000000000000, 0.000000000000000000, -0.000000000000000000 ) ) ;
#11868=COLOUR_RGB('Light Blue',0.38,0.62,0.78);
#11869=FILL_AREA_STYLE_COLOUR('',#11868);
#11870=FILL_AREA_STYLE('',(#11869));
#11871=SURFACE_STYLE_FILL_AREA(#11870);
#11872=SURFACE_SIDE_STYLE('',(#11871));
#11873=SURFACE_STYLE_USAGE(.BOTH.,#11872);
#11874=PRESENTATION_STYLE_ASSIGNMENT((#11873));
ENDSEC;
END-ISO-10303-21;
